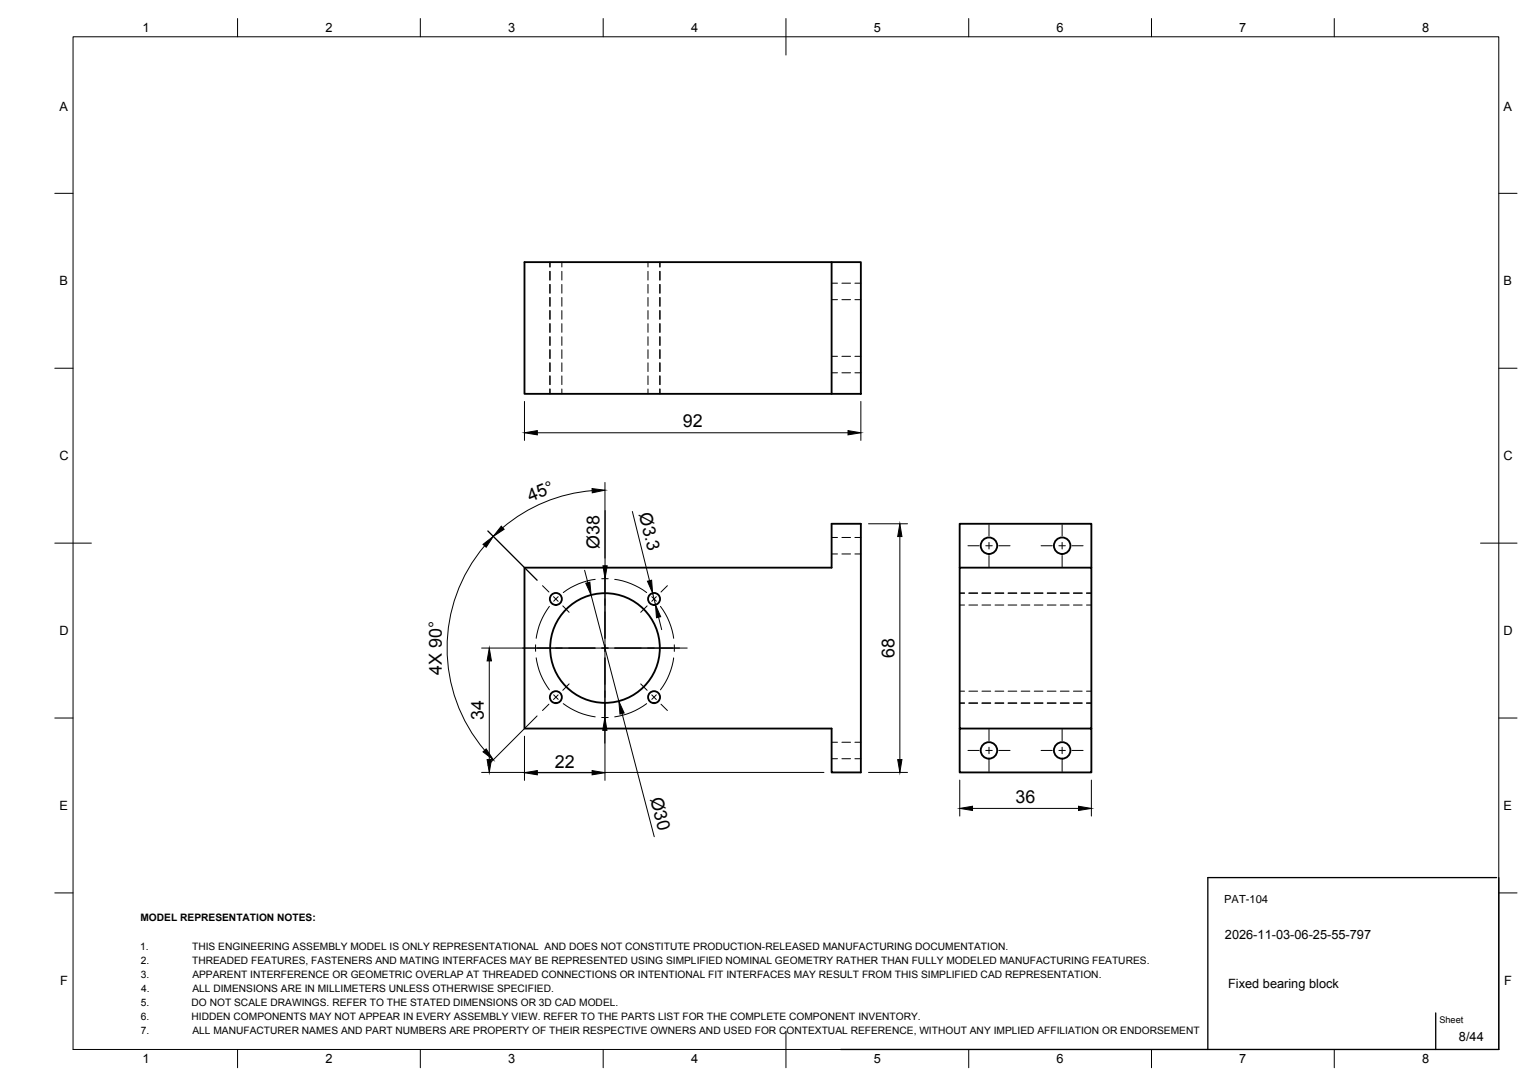
ISO-10303-21;
HEADER;
/* Generated by software containing ST-Developer
 * from STEP Tools, Inc. (www.steptools.com) 
 */

FILE_DESCRIPTION(
/* description */ ('Timing belt drive module 2 mm Pitch Timing 20T-40T'),

/* implementation_level */ '2;1');

FILE_NAME(
/* name */ 'Fixed bearing block.step',
/* time_stamp */ '2026-10-28T03:25:12-07:00',
/* author */ (''),
/* organization */ (''),
/* preprocessor_version */ 'ST-DEVELOPER v20.2',
/* originating_system */ 'Autodesk Translation Framework v15.17.0.0',
/* authorisation */ '');

FILE_SCHEMA (('AUTOMOTIVE_DESIGN { 1 0 10303 214 3 1 1 }'));
ENDSEC;

DATA;
#10=MECHANICAL_DESIGN_GEOMETRIC_PRESENTATION_REPRESENTATION('',(#527),#17830);
#441=SHAPE_REPRESENTATION_RELATIONSHIP('SRR','None',#18011,#484);
#484=ADVANCED_BREP_SHAPE_REPRESENTATION('',(#585),#17786);
#527=STYLED_ITEM('',(#18317),#585);
#585=MANIFOLD_SOLID_BREP('Body1',#8984);
#647=FACE_BOUND('',#1545,.T.);
#648=FACE_BOUND('',#1546,.T.);
#649=FACE_BOUND('',#1548,.T.);
#650=FACE_BOUND('',#1549,.T.);
#651=FACE_BOUND('',#1553,.T.);
#652=FACE_BOUND('',#1554,.T.);
#653=FACE_BOUND('',#1555,.T.);
#654=FACE_BOUND('',#1556,.T.);
#655=FACE_BOUND('',#1557,.T.);
#656=FACE_BOUND('',#1560,.T.);
#657=FACE_BOUND('',#1561,.T.);
#658=FACE_BOUND('',#1562,.T.);
#659=FACE_BOUND('',#1563,.T.);
#660=FACE_BOUND('',#1564,.T.);
#661=FACE_BOUND('',#1568,.T.);
#662=FACE_BOUND('',#1569,.T.);
#663=FACE_BOUND('',#1570,.T.);
#664=FACE_BOUND('',#1571,.T.);
#803=PLANE('',#9619);
#804=PLANE('',#9620);
#805=PLANE('',#9621);
#806=PLANE('',#9622);
#807=PLANE('',#9623);
#808=PLANE('',#9624);
#809=PLANE('',#9625);
#810=PLANE('',#9626);
#811=PLANE('',#9627);
#812=PLANE('',#9628);
#1004=FACE_OUTER_BOUND('',#1535,.T.);
#1005=FACE_OUTER_BOUND('',#1536,.T.);
#1006=FACE_OUTER_BOUND('',#1537,.T.);
#1007=FACE_OUTER_BOUND('',#1538,.T.);
#1008=FACE_OUTER_BOUND('',#1539,.T.);
#1009=FACE_OUTER_BOUND('',#1540,.T.);
#1010=FACE_OUTER_BOUND('',#1541,.T.);
#1011=FACE_OUTER_BOUND('',#1542,.T.);
#1012=FACE_OUTER_BOUND('',#1543,.T.);
#1013=FACE_OUTER_BOUND('',#1544,.T.);
#1014=FACE_OUTER_BOUND('',#1547,.T.);
#1015=FACE_OUTER_BOUND('',#1550,.T.);
#1016=FACE_OUTER_BOUND('',#1551,.T.);
#1017=FACE_OUTER_BOUND('',#1552,.T.);
#1018=FACE_OUTER_BOUND('',#1558,.T.);
#1019=FACE_OUTER_BOUND('',#1559,.T.);
#1020=FACE_OUTER_BOUND('',#1565,.T.);
#1021=FACE_OUTER_BOUND('',#1566,.T.);
#1022=FACE_OUTER_BOUND('',#1567,.T.);
#1535=EDGE_LOOP('',(#5977,#5978,#5979,#5980));
#1536=EDGE_LOOP('',(#5981,#5982,#5983,#5984));
#1537=EDGE_LOOP('',(#5985,#5986,#5987,#5988));
#1538=EDGE_LOOP('',(#5989,#5990,#5991,#5992));
#1539=EDGE_LOOP('',(#5993,#5994,#5995,#5996));
#1540=EDGE_LOOP('',(#5997,#5998,#5999,#6000));
#1541=EDGE_LOOP('',(#6001,#6002,#6003,#6004));
#1542=EDGE_LOOP('',(#6005,#6006,#6007,#6008));
#1543=EDGE_LOOP('',(#6009,#6010,#6011,#6012));
#1544=EDGE_LOOP('',(#6013,#6014,#6015,#6016));
#1545=EDGE_LOOP('',(#6017));
#1546=EDGE_LOOP('',(#6018));
#1547=EDGE_LOOP('',(#6019,#6020,#6021,#6022));
#1548=EDGE_LOOP('',(#6023));
#1549=EDGE_LOOP('',(#6024));
#1550=EDGE_LOOP('',(#6025,#6026,#6027,#6028));
#1551=EDGE_LOOP('',(#6029,#6030,#6031,#6032));
#1552=EDGE_LOOP('',(#6033,#6034,#6035,#6036,#6037,#6038,#6039,#6040));
#1553=EDGE_LOOP('',(#6041));
#1554=EDGE_LOOP('',(#6042));
#1555=EDGE_LOOP('',(#6043));
#1556=EDGE_LOOP('',(#6044));
#1557=EDGE_LOOP('',(#6045));
#1558=EDGE_LOOP('',(#6046,#6047,#6048,#6049));
#1559=EDGE_LOOP('',(#6050,#6051,#6052,#6053,#6054,#6055,#6056,#6057));
#1560=EDGE_LOOP('',(#6058));
#1561=EDGE_LOOP('',(#6059));
#1562=EDGE_LOOP('',(#6060));
#1563=EDGE_LOOP('',(#6061));
#1564=EDGE_LOOP('',(#6062));
#1565=EDGE_LOOP('',(#6063,#6064,#6065,#6066));
#1566=EDGE_LOOP('',(#6067,#6068,#6069,#6070));
#1567=EDGE_LOOP('',(#6071,#6072,#6073,#6074));
#1568=EDGE_LOOP('',(#6075));
#1569=EDGE_LOOP('',(#6076));
#1570=EDGE_LOOP('',(#6077));
#1571=EDGE_LOOP('',(#6078));
#2168=CIRCLE('',#9593,0.165);
#2169=CIRCLE('',#9594,0.165);
#2170=CIRCLE('',#9596,0.165);
#2171=CIRCLE('',#9597,0.165);
#2172=CIRCLE('',#9599,0.165);
#2173=CIRCLE('',#9600,0.165);
#2174=CIRCLE('',#9602,0.165);
#2175=CIRCLE('',#9603,0.165);
#2176=CIRCLE('',#9605,1.5);
#2177=CIRCLE('',#9606,1.5);
#2178=CIRCLE('',#9608,0.225);
#2179=CIRCLE('',#9609,0.225);
#2180=CIRCLE('',#9611,0.225);
#2181=CIRCLE('',#9612,0.225);
#2182=CIRCLE('',#9614,0.225);
#2183=CIRCLE('',#9615,0.225);
#2184=CIRCLE('',#9617,0.225);
#2185=CIRCLE('',#9618,0.225);
#2864=LINE('',#14095,#3342);
#2865=LINE('',#14101,#3343);
#2866=LINE('',#14107,#3344);
#2867=LINE('',#14113,#3345);
#2868=LINE('',#14119,#3346);
#2869=LINE('',#14125,#3347);
#2870=LINE('',#14131,#3348);
#2871=LINE('',#14137,#3349);
#2872=LINE('',#14143,#3350);
#2873=LINE('',#14148,#3351);
#2874=LINE('',#14150,#3352);
#2875=LINE('',#14152,#3353);
#2876=LINE('',#14153,#3354);
#2877=LINE('',#14157,#3355);
#2878=LINE('',#14159,#3356);
#2879=LINE('',#14161,#3357);
#2880=LINE('',#14162,#3358);
#2881=LINE('',#14165,#3359);
#2882=LINE('',#14167,#3360);
#2883=LINE('',#14168,#3361);
#2884=LINE('',#14171,#3362);
#2885=LINE('',#14173,#3363);
#2886=LINE('',#14174,#3364);
#2887=LINE('',#14177,#3365);
#2888=LINE('',#14179,#3366);
#2889=LINE('',#14180,#3367);
#2890=LINE('',#14181,#3368);
#2891=LINE('',#14184,#3369);
#2892=LINE('',#14185,#3370);
#2893=LINE('',#14188,#3371);
#2894=LINE('',#14189,#3372);
#2895=LINE('',#14190,#3373);
#2896=LINE('',#14192,#3374);
#3342=VECTOR('',#11039,0.165);
#3343=VECTOR('',#11046,0.165);
#3344=VECTOR('',#11053,0.165);
#3345=VECTOR('',#11060,0.165);
#3346=VECTOR('',#11067,1.5);
#3347=VECTOR('',#11074,0.225);
#3348=VECTOR('',#11081,0.225);
#3349=VECTOR('',#11088,0.225);
#3350=VECTOR('',#11095,0.225);
#3351=VECTOR('',#11100,1.);
#3352=VECTOR('',#11101,1.);
#3353=VECTOR('',#11102,1.);
#3354=VECTOR('',#11103,1.);
#3355=VECTOR('',#11106,1.);
#3356=VECTOR('',#11107,1.);
#3357=VECTOR('',#11108,1.);
#3358=VECTOR('',#11109,1.);
#3359=VECTOR('',#11112,1.);
#3360=VECTOR('',#11113,1.);
#3361=VECTOR('',#11114,1.);
#3362=VECTOR('',#11117,1.);
#3363=VECTOR('',#11118,1.);
#3364=VECTOR('',#11119,1.);
#3365=VECTOR('',#11122,1.);
#3366=VECTOR('',#11123,1.);
#3367=VECTOR('',#11124,1.);
#3368=VECTOR('',#11125,1.);
#3369=VECTOR('',#11128,1.);
#3370=VECTOR('',#11129,1.);
#3371=VECTOR('',#11132,1.);
#3372=VECTOR('',#11133,1.);
#3373=VECTOR('',#11134,1.);
#3374=VECTOR('',#11137,1.);
#3814=VERTEX_POINT('',#14092);
#3815=VERTEX_POINT('',#14094);
#3816=VERTEX_POINT('',#14098);
#3817=VERTEX_POINT('',#14100);
#3818=VERTEX_POINT('',#14104);
#3819=VERTEX_POINT('',#14106);
#3820=VERTEX_POINT('',#14110);
#3821=VERTEX_POINT('',#14112);
#3822=VERTEX_POINT('',#14116);
#3823=VERTEX_POINT('',#14118);
#3824=VERTEX_POINT('',#14122);
#3825=VERTEX_POINT('',#14124);
#3826=VERTEX_POINT('',#14128);
#3827=VERTEX_POINT('',#14130);
#3828=VERTEX_POINT('',#14134);
#3829=VERTEX_POINT('',#14136);
#3830=VERTEX_POINT('',#14140);
#3831=VERTEX_POINT('',#14142);
#3832=VERTEX_POINT('',#14146);
#3833=VERTEX_POINT('',#14147);
#3834=VERTEX_POINT('',#14149);
#3835=VERTEX_POINT('',#14151);
#3836=VERTEX_POINT('',#14155);
#3837=VERTEX_POINT('',#14156);
#3838=VERTEX_POINT('',#14158);
#3839=VERTEX_POINT('',#14160);
#3840=VERTEX_POINT('',#14164);
#3841=VERTEX_POINT('',#14166);
#3842=VERTEX_POINT('',#14170);
#3843=VERTEX_POINT('',#14172);
#3844=VERTEX_POINT('',#14176);
#3845=VERTEX_POINT('',#14178);
#3846=VERTEX_POINT('',#14183);
#3847=VERTEX_POINT('',#14187);
#4671=EDGE_CURVE('',#3814,#3814,#2168,.T.);
#4672=EDGE_CURVE('',#3814,#3815,#2864,.T.);
#4673=EDGE_CURVE('',#3815,#3815,#2169,.T.);
#4674=EDGE_CURVE('',#3816,#3816,#2170,.T.);
#4675=EDGE_CURVE('',#3816,#3817,#2865,.T.);
#4676=EDGE_CURVE('',#3817,#3817,#2171,.T.);
#4677=EDGE_CURVE('',#3818,#3818,#2172,.T.);
#4678=EDGE_CURVE('',#3818,#3819,#2866,.T.);
#4679=EDGE_CURVE('',#3819,#3819,#2173,.T.);
#4680=EDGE_CURVE('',#3820,#3820,#2174,.T.);
#4681=EDGE_CURVE('',#3820,#3821,#2867,.T.);
#4682=EDGE_CURVE('',#3821,#3821,#2175,.T.);
#4683=EDGE_CURVE('',#3822,#3822,#2176,.T.);
#4684=EDGE_CURVE('',#3822,#3823,#2868,.T.);
#4685=EDGE_CURVE('',#3823,#3823,#2177,.T.);
#4686=EDGE_CURVE('',#3824,#3824,#2178,.T.);
#4687=EDGE_CURVE('',#3824,#3825,#2869,.T.);
#4688=EDGE_CURVE('',#3825,#3825,#2179,.T.);
#4689=EDGE_CURVE('',#3826,#3826,#2180,.T.);
#4690=EDGE_CURVE('',#3826,#3827,#2870,.T.);
#4691=EDGE_CURVE('',#3827,#3827,#2181,.T.);
#4692=EDGE_CURVE('',#3828,#3828,#2182,.T.);
#4693=EDGE_CURVE('',#3828,#3829,#2871,.T.);
#4694=EDGE_CURVE('',#3829,#3829,#2183,.T.);
#4695=EDGE_CURVE('',#3830,#3830,#2184,.T.);
#4696=EDGE_CURVE('',#3830,#3831,#2872,.T.);
#4697=EDGE_CURVE('',#3831,#3831,#2185,.T.);
#4698=EDGE_CURVE('',#3832,#3833,#2873,.T.);
#4699=EDGE_CURVE('',#3834,#3832,#2874,.T.);
#4700=EDGE_CURVE('',#3834,#3835,#2875,.T.);
#4701=EDGE_CURVE('',#3833,#3835,#2876,.T.);
#4702=EDGE_CURVE('',#3836,#3837,#2877,.T.);
#4703=EDGE_CURVE('',#3838,#3836,#2878,.T.);
#4704=EDGE_CURVE('',#3839,#3838,#2879,.T.);
#4705=EDGE_CURVE('',#3837,#3839,#2880,.T.);
#4706=EDGE_CURVE('',#3839,#3840,#2881,.T.);
#4707=EDGE_CURVE('',#3841,#3838,#2882,.T.);
#4708=EDGE_CURVE('',#3840,#3841,#2883,.T.);
#4709=EDGE_CURVE('',#3842,#3834,#2884,.T.);
#4710=EDGE_CURVE('',#3842,#3843,#2885,.T.);
#4711=EDGE_CURVE('',#3835,#3843,#2886,.T.);
#4712=EDGE_CURVE('',#3832,#3844,#2887,.T.);
#4713=EDGE_CURVE('',#3845,#3844,#2888,.T.);
#4714=EDGE_CURVE('',#3837,#3845,#2889,.T.);
#4715=EDGE_CURVE('',#3840,#3842,#2890,.T.);
#4716=EDGE_CURVE('',#3833,#3846,#2891,.T.);
#4717=EDGE_CURVE('',#3844,#3846,#2892,.T.);
#4718=EDGE_CURVE('',#3836,#3847,#2893,.T.);
#4719=EDGE_CURVE('',#3846,#3847,#2894,.T.);
#4720=EDGE_CURVE('',#3843,#3841,#2895,.T.);
#4721=EDGE_CURVE('',#3847,#3845,#2896,.T.);
#5977=ORIENTED_EDGE('',*,*,#4671,.F.);
#5978=ORIENTED_EDGE('',*,*,#4672,.T.);
#5979=ORIENTED_EDGE('',*,*,#4673,.F.);
#5980=ORIENTED_EDGE('',*,*,#4672,.F.);
#5981=ORIENTED_EDGE('',*,*,#4674,.F.);
#5982=ORIENTED_EDGE('',*,*,#4675,.T.);
#5983=ORIENTED_EDGE('',*,*,#4676,.F.);
#5984=ORIENTED_EDGE('',*,*,#4675,.F.);
#5985=ORIENTED_EDGE('',*,*,#4677,.F.);
#5986=ORIENTED_EDGE('',*,*,#4678,.T.);
#5987=ORIENTED_EDGE('',*,*,#4679,.F.);
#5988=ORIENTED_EDGE('',*,*,#4678,.F.);
#5989=ORIENTED_EDGE('',*,*,#4680,.F.);
#5990=ORIENTED_EDGE('',*,*,#4681,.T.);
#5991=ORIENTED_EDGE('',*,*,#4682,.F.);
#5992=ORIENTED_EDGE('',*,*,#4681,.F.);
#5993=ORIENTED_EDGE('',*,*,#4683,.F.);
#5994=ORIENTED_EDGE('',*,*,#4684,.T.);
#5995=ORIENTED_EDGE('',*,*,#4685,.F.);
#5996=ORIENTED_EDGE('',*,*,#4684,.F.);
#5997=ORIENTED_EDGE('',*,*,#4686,.F.);
#5998=ORIENTED_EDGE('',*,*,#4687,.T.);
#5999=ORIENTED_EDGE('',*,*,#4688,.F.);
#6000=ORIENTED_EDGE('',*,*,#4687,.F.);
#6001=ORIENTED_EDGE('',*,*,#4689,.F.);
#6002=ORIENTED_EDGE('',*,*,#4690,.T.);
#6003=ORIENTED_EDGE('',*,*,#4691,.F.);
#6004=ORIENTED_EDGE('',*,*,#4690,.F.);
#6005=ORIENTED_EDGE('',*,*,#4692,.F.);
#6006=ORIENTED_EDGE('',*,*,#4693,.T.);
#6007=ORIENTED_EDGE('',*,*,#4694,.F.);
#6008=ORIENTED_EDGE('',*,*,#4693,.F.);
#6009=ORIENTED_EDGE('',*,*,#4695,.F.);
#6010=ORIENTED_EDGE('',*,*,#4696,.T.);
#6011=ORIENTED_EDGE('',*,*,#4697,.F.);
#6012=ORIENTED_EDGE('',*,*,#4696,.F.);
#6013=ORIENTED_EDGE('',*,*,#4698,.F.);
#6014=ORIENTED_EDGE('',*,*,#4699,.F.);
#6015=ORIENTED_EDGE('',*,*,#4700,.T.);
#6016=ORIENTED_EDGE('',*,*,#4701,.F.);
#6017=ORIENTED_EDGE('',*,*,#4688,.T.);
#6018=ORIENTED_EDGE('',*,*,#4697,.T.);
#6019=ORIENTED_EDGE('',*,*,#4702,.F.);
#6020=ORIENTED_EDGE('',*,*,#4703,.F.);
#6021=ORIENTED_EDGE('',*,*,#4704,.F.);
#6022=ORIENTED_EDGE('',*,*,#4705,.F.);
#6023=ORIENTED_EDGE('',*,*,#4691,.T.);
#6024=ORIENTED_EDGE('',*,*,#4694,.T.);
#6025=ORIENTED_EDGE('',*,*,#4706,.F.);
#6026=ORIENTED_EDGE('',*,*,#4704,.T.);
#6027=ORIENTED_EDGE('',*,*,#4707,.F.);
#6028=ORIENTED_EDGE('',*,*,#4708,.F.);
#6029=ORIENTED_EDGE('',*,*,#4709,.F.);
#6030=ORIENTED_EDGE('',*,*,#4710,.T.);
#6031=ORIENTED_EDGE('',*,*,#4711,.F.);
#6032=ORIENTED_EDGE('',*,*,#4700,.F.);
#6033=ORIENTED_EDGE('',*,*,#4712,.T.);
#6034=ORIENTED_EDGE('',*,*,#4713,.F.);
#6035=ORIENTED_EDGE('',*,*,#4714,.F.);
#6036=ORIENTED_EDGE('',*,*,#4705,.T.);
#6037=ORIENTED_EDGE('',*,*,#4706,.T.);
#6038=ORIENTED_EDGE('',*,*,#4715,.T.);
#6039=ORIENTED_EDGE('',*,*,#4709,.T.);
#6040=ORIENTED_EDGE('',*,*,#4699,.T.);
#6041=ORIENTED_EDGE('',*,*,#4683,.T.);
#6042=ORIENTED_EDGE('',*,*,#4680,.T.);
#6043=ORIENTED_EDGE('',*,*,#4677,.T.);
#6044=ORIENTED_EDGE('',*,*,#4674,.T.);
#6045=ORIENTED_EDGE('',*,*,#4671,.T.);
#6046=ORIENTED_EDGE('',*,*,#4698,.T.);
#6047=ORIENTED_EDGE('',*,*,#4716,.T.);
#6048=ORIENTED_EDGE('',*,*,#4717,.F.);
#6049=ORIENTED_EDGE('',*,*,#4712,.F.);
#6050=ORIENTED_EDGE('',*,*,#4718,.T.);
#6051=ORIENTED_EDGE('',*,*,#4719,.F.);
#6052=ORIENTED_EDGE('',*,*,#4716,.F.);
#6053=ORIENTED_EDGE('',*,*,#4701,.T.);
#6054=ORIENTED_EDGE('',*,*,#4711,.T.);
#6055=ORIENTED_EDGE('',*,*,#4720,.T.);
#6056=ORIENTED_EDGE('',*,*,#4707,.T.);
#6057=ORIENTED_EDGE('',*,*,#4703,.T.);
#6058=ORIENTED_EDGE('',*,*,#4685,.T.);
#6059=ORIENTED_EDGE('',*,*,#4682,.T.);
#6060=ORIENTED_EDGE('',*,*,#4679,.T.);
#6061=ORIENTED_EDGE('',*,*,#4676,.T.);
#6062=ORIENTED_EDGE('',*,*,#4673,.T.);
#6063=ORIENTED_EDGE('',*,*,#4702,.T.);
#6064=ORIENTED_EDGE('',*,*,#4714,.T.);
#6065=ORIENTED_EDGE('',*,*,#4721,.F.);
#6066=ORIENTED_EDGE('',*,*,#4718,.F.);
#6067=ORIENTED_EDGE('',*,*,#4721,.T.);
#6068=ORIENTED_EDGE('',*,*,#4713,.T.);
#6069=ORIENTED_EDGE('',*,*,#4717,.T.);
#6070=ORIENTED_EDGE('',*,*,#4719,.T.);
#6071=ORIENTED_EDGE('',*,*,#4720,.F.);
#6072=ORIENTED_EDGE('',*,*,#4710,.F.);
#6073=ORIENTED_EDGE('',*,*,#4715,.F.);
#6074=ORIENTED_EDGE('',*,*,#4708,.T.);
#6075=ORIENTED_EDGE('',*,*,#4686,.T.);
#6076=ORIENTED_EDGE('',*,*,#4689,.T.);
#6077=ORIENTED_EDGE('',*,*,#4692,.T.);
#6078=ORIENTED_EDGE('',*,*,#4695,.T.);
#8193=CYLINDRICAL_SURFACE('',#9592,0.165);
#8194=CYLINDRICAL_SURFACE('',#9595,0.165);
#8195=CYLINDRICAL_SURFACE('',#9598,0.165);
#8196=CYLINDRICAL_SURFACE('',#9601,0.165);
#8197=CYLINDRICAL_SURFACE('',#9604,1.5);
#8198=CYLINDRICAL_SURFACE('',#9607,0.225);
#8199=CYLINDRICAL_SURFACE('',#9610,0.225);
#8200=CYLINDRICAL_SURFACE('',#9613,0.225);
#8201=CYLINDRICAL_SURFACE('',#9616,0.225);
#8502=ADVANCED_FACE('',(#1004),#8193,.F.);
#8503=ADVANCED_FACE('',(#1005),#8194,.F.);
#8504=ADVANCED_FACE('',(#1006),#8195,.F.);
#8505=ADVANCED_FACE('',(#1007),#8196,.F.);
#8506=ADVANCED_FACE('',(#1008),#8197,.F.);
#8507=ADVANCED_FACE('',(#1009),#8198,.F.);
#8508=ADVANCED_FACE('',(#1010),#8199,.F.);
#8509=ADVANCED_FACE('',(#1011),#8200,.F.);
#8510=ADVANCED_FACE('',(#1012),#8201,.F.);
#8511=ADVANCED_FACE('',(#1013,#647,#648),#803,.T.);
#8512=ADVANCED_FACE('',(#1014,#649,#650),#804,.T.);
#8513=ADVANCED_FACE('',(#1015),#805,.T.);
#8514=ADVANCED_FACE('',(#1016),#806,.T.);
#8515=ADVANCED_FACE('',(#1017,#651,#652,#653,#654,#655),#807,.T.);
#8516=ADVANCED_FACE('',(#1018),#808,.T.);
#8517=ADVANCED_FACE('',(#1019,#656,#657,#658,#659,#660),#809,.T.);
#8518=ADVANCED_FACE('',(#1020),#810,.T.);
#8519=ADVANCED_FACE('',(#1021),#811,.T.);
#8520=ADVANCED_FACE('',(#1022,#661,#662,#663,#664),#812,.F.);
#8984=CLOSED_SHELL('',(#8502,#8503,#8504,#8505,#8506,#8507,#8508,#8509,
#8510,#8511,#8512,#8513,#8514,#8515,#8516,#8517,#8518,#8519,#8520));
#9591=AXIS2_PLACEMENT_3D('',#14090,#11033,#11034);
#9592=AXIS2_PLACEMENT_3D('',#14091,#11035,#11036);
#9593=AXIS2_PLACEMENT_3D('',#14093,#11037,#11038);
#9594=AXIS2_PLACEMENT_3D('',#14096,#11040,#11041);
#9595=AXIS2_PLACEMENT_3D('',#14097,#11042,#11043);
#9596=AXIS2_PLACEMENT_3D('',#14099,#11044,#11045);
#9597=AXIS2_PLACEMENT_3D('',#14102,#11047,#11048);
#9598=AXIS2_PLACEMENT_3D('',#14103,#11049,#11050);
#9599=AXIS2_PLACEMENT_3D('',#14105,#11051,#11052);
#9600=AXIS2_PLACEMENT_3D('',#14108,#11054,#11055);
#9601=AXIS2_PLACEMENT_3D('',#14109,#11056,#11057);
#9602=AXIS2_PLACEMENT_3D('',#14111,#11058,#11059);
#9603=AXIS2_PLACEMENT_3D('',#14114,#11061,#11062);
#9604=AXIS2_PLACEMENT_3D('',#14115,#11063,#11064);
#9605=AXIS2_PLACEMENT_3D('',#14117,#11065,#11066);
#9606=AXIS2_PLACEMENT_3D('',#14120,#11068,#11069);
#9607=AXIS2_PLACEMENT_3D('',#14121,#11070,#11071);
#9608=AXIS2_PLACEMENT_3D('',#14123,#11072,#11073);
#9609=AXIS2_PLACEMENT_3D('',#14126,#11075,#11076);
#9610=AXIS2_PLACEMENT_3D('',#14127,#11077,#11078);
#9611=AXIS2_PLACEMENT_3D('',#14129,#11079,#11080);
#9612=AXIS2_PLACEMENT_3D('',#14132,#11082,#11083);
#9613=AXIS2_PLACEMENT_3D('',#14133,#11084,#11085);
#9614=AXIS2_PLACEMENT_3D('',#14135,#11086,#11087);
#9615=AXIS2_PLACEMENT_3D('',#14138,#11089,#11090);
#9616=AXIS2_PLACEMENT_3D('',#14139,#11091,#11092);
#9617=AXIS2_PLACEMENT_3D('',#14141,#11093,#11094);
#9618=AXIS2_PLACEMENT_3D('',#14144,#11096,#11097);
#9619=AXIS2_PLACEMENT_3D('',#14145,#11098,#11099);
#9620=AXIS2_PLACEMENT_3D('',#14154,#11104,#11105);
#9621=AXIS2_PLACEMENT_3D('',#14163,#11110,#11111);
#9622=AXIS2_PLACEMENT_3D('',#14169,#11115,#11116);
#9623=AXIS2_PLACEMENT_3D('',#14175,#11120,#11121);
#9624=AXIS2_PLACEMENT_3D('',#14182,#11126,#11127);
#9625=AXIS2_PLACEMENT_3D('',#14186,#11130,#11131);
#9626=AXIS2_PLACEMENT_3D('',#14191,#11135,#11136);
#9627=AXIS2_PLACEMENT_3D('',#14193,#11138,#11139);
#9628=AXIS2_PLACEMENT_3D('',#14194,#11140,#11141);
#11033=DIRECTION('axis',(0.,0.,1.));
#11034=DIRECTION('refdir',(1.,0.,0.));
#11035=DIRECTION('center_axis',(0.,1.,0.));
#11036=DIRECTION('ref_axis',(1.,0.,0.));
#11037=DIRECTION('center_axis',(0.,1.,0.));
#11038=DIRECTION('ref_axis',(1.,0.,0.));
#11039=DIRECTION('',(0.,1.,0.));
#11040=DIRECTION('center_axis',(0.,-1.,0.));
#11041=DIRECTION('ref_axis',(1.,0.,0.));
#11042=DIRECTION('center_axis',(0.,1.,0.));
#11043=DIRECTION('ref_axis',(1.,0.,0.));
#11044=DIRECTION('center_axis',(0.,1.,0.));
#11045=DIRECTION('ref_axis',(1.,0.,0.));
#11046=DIRECTION('',(0.,1.,0.));
#11047=DIRECTION('center_axis',(0.,-1.,0.));
#11048=DIRECTION('ref_axis',(1.,0.,0.));
#11049=DIRECTION('center_axis',(0.,1.,0.));
#11050=DIRECTION('ref_axis',(1.,0.,0.));
#11051=DIRECTION('center_axis',(0.,1.,0.));
#11052=DIRECTION('ref_axis',(1.,0.,0.));
#11053=DIRECTION('',(0.,1.,0.));
#11054=DIRECTION('center_axis',(0.,-1.,0.));
#11055=DIRECTION('ref_axis',(1.,0.,0.));
#11056=DIRECTION('center_axis',(0.,1.,0.));
#11057=DIRECTION('ref_axis',(1.,0.,0.));
#11058=DIRECTION('center_axis',(0.,1.,0.));
#11059=DIRECTION('ref_axis',(1.,0.,0.));
#11060=DIRECTION('',(0.,1.,0.));
#11061=DIRECTION('center_axis',(0.,-1.,0.));
#11062=DIRECTION('ref_axis',(1.,0.,0.));
#11063=DIRECTION('center_axis',(0.,1.,0.));
#11064=DIRECTION('ref_axis',(1.,0.,0.));
#11065=DIRECTION('center_axis',(0.,1.,0.));
#11066=DIRECTION('ref_axis',(1.,0.,0.));
#11067=DIRECTION('',(0.,1.,0.));
#11068=DIRECTION('center_axis',(0.,-1.,0.));
#11069=DIRECTION('ref_axis',(1.,0.,0.));
#11070=DIRECTION('center_axis',(0.,0.,1.));
#11071=DIRECTION('ref_axis',(1.,0.,0.));
#11072=DIRECTION('center_axis',(0.,0.,1.));
#11073=DIRECTION('ref_axis',(1.,0.,0.));
#11074=DIRECTION('',(0.,0.,1.));
#11075=DIRECTION('center_axis',(0.,0.,-1.));
#11076=DIRECTION('ref_axis',(1.,0.,0.));
#11077=DIRECTION('center_axis',(0.,0.,1.));
#11078=DIRECTION('ref_axis',(1.,0.,0.));
#11079=DIRECTION('center_axis',(0.,0.,1.));
#11080=DIRECTION('ref_axis',(1.,0.,0.));
#11081=DIRECTION('',(0.,0.,1.));
#11082=DIRECTION('center_axis',(0.,0.,-1.));
#11083=DIRECTION('ref_axis',(1.,0.,0.));
#11084=DIRECTION('center_axis',(0.,0.,1.));
#11085=DIRECTION('ref_axis',(1.,0.,0.));
#11086=DIRECTION('center_axis',(0.,0.,1.));
#11087=DIRECTION('ref_axis',(1.,0.,0.));
#11088=DIRECTION('',(0.,0.,1.));
#11089=DIRECTION('center_axis',(0.,0.,-1.));
#11090=DIRECTION('ref_axis',(1.,0.,0.));
#11091=DIRECTION('center_axis',(0.,0.,1.));
#11092=DIRECTION('ref_axis',(1.,0.,0.));
#11093=DIRECTION('center_axis',(0.,0.,1.));
#11094=DIRECTION('ref_axis',(1.,0.,0.));
#11095=DIRECTION('',(0.,0.,1.));
#11096=DIRECTION('center_axis',(0.,0.,-1.));
#11097=DIRECTION('ref_axis',(1.,0.,0.));
#11098=DIRECTION('center_axis',(0.,0.,1.));
#11099=DIRECTION('ref_axis',(1.,0.,0.));
#11100=DIRECTION('',(0.,1.,0.));
#11101=DIRECTION('',(-1.,0.,0.));
#11102=DIRECTION('',(0.,1.,0.));
#11103=DIRECTION('',(1.,0.,0.));
#11104=DIRECTION('center_axis',(0.,0.,1.));
#11105=DIRECTION('ref_axis',(1.,0.,0.));
#11106=DIRECTION('',(0.,-1.,0.));
#11107=DIRECTION('',(1.,0.,0.));
#11108=DIRECTION('',(0.,1.,0.));
#11109=DIRECTION('',(-1.,0.,0.));
#11110=DIRECTION('center_axis',(-1.,0.,0.));
#11111=DIRECTION('ref_axis',(0.,0.,1.));
#11112=DIRECTION('',(0.,0.,-1.));
#11113=DIRECTION('',(0.,0.,1.));
#11114=DIRECTION('',(0.,1.,0.));
#11115=DIRECTION('center_axis',(1.,0.,0.));
#11116=DIRECTION('ref_axis',(0.,0.,-1.));
#11117=DIRECTION('',(0.,0.,1.));
#11118=DIRECTION('',(0.,1.,0.));
#11119=DIRECTION('',(0.,0.,-1.));
#11120=DIRECTION('center_axis',(0.,-1.,0.));
#11121=DIRECTION('ref_axis',(1.,0.,0.));
#11122=DIRECTION('',(0.,0.,1.));
#11123=DIRECTION('',(1.,0.,0.));
#11124=DIRECTION('',(0.,0.,1.));
#11125=DIRECTION('',(1.,0.,0.));
#11126=DIRECTION('center_axis',(1.,0.,0.));
#11127=DIRECTION('ref_axis',(0.,1.,0.));
#11128=DIRECTION('',(0.,0.,1.));
#11129=DIRECTION('',(0.,1.,0.));
#11130=DIRECTION('center_axis',(0.,1.,0.));
#11131=DIRECTION('ref_axis',(-1.,0.,0.));
#11132=DIRECTION('',(0.,0.,1.));
#11133=DIRECTION('',(-1.,0.,0.));
#11134=DIRECTION('',(-1.,0.,0.));
#11135=DIRECTION('center_axis',(-1.,0.,0.));
#11136=DIRECTION('ref_axis',(0.,-1.,0.));
#11137=DIRECTION('',(0.,-1.,0.));
#11138=DIRECTION('center_axis',(0.,0.,1.));
#11139=DIRECTION('ref_axis',(1.,0.,0.));
#11140=DIRECTION('center_axis',(0.,0.,1.));
#11141=DIRECTION('ref_axis',(1.,0.,0.));
#14090=CARTESIAN_POINT('',(0.,0.,0.));
#14091=CARTESIAN_POINT('Origin',(-1.34350288425444,-1.9,5.65649711574556));
#14092=CARTESIAN_POINT('',(-1.50850288425444,-1.8,5.65649711574556));
#14093=CARTESIAN_POINT('Origin',(-1.34350288425444,-1.8,5.65649711574556));
#14094=CARTESIAN_POINT('',(-1.50850288425444,1.8,5.65649711574556));
#14095=CARTESIAN_POINT('',(-1.50850288425444,-1.9,5.65649711574556));
#14096=CARTESIAN_POINT('Origin',(-1.34350288425444,1.8,5.65649711574556));
#14097=CARTESIAN_POINT('Origin',(-1.34350288425444,-1.9,8.34350288425444));
#14098=CARTESIAN_POINT('',(-1.50850288425444,-1.8,8.34350288425444));
#14099=CARTESIAN_POINT('Origin',(-1.34350288425444,-1.8,8.34350288425444));
#14100=CARTESIAN_POINT('',(-1.50850288425444,1.8,8.34350288425444));
#14101=CARTESIAN_POINT('',(-1.50850288425444,-1.9,8.34350288425444));
#14102=CARTESIAN_POINT('Origin',(-1.34350288425444,1.8,8.34350288425444));
#14103=CARTESIAN_POINT('Origin',(1.34350288425444,-1.9,8.34350288425444));
#14104=CARTESIAN_POINT('',(1.17850288425444,-1.8,8.34350288425444));
#14105=CARTESIAN_POINT('Origin',(1.34350288425444,-1.8,8.34350288425444));
#14106=CARTESIAN_POINT('',(1.17850288425444,1.8,8.34350288425444));
#14107=CARTESIAN_POINT('',(1.17850288425444,-1.9,8.34350288425444));
#14108=CARTESIAN_POINT('Origin',(1.34350288425444,1.8,8.34350288425444));
#14109=CARTESIAN_POINT('Origin',(1.34350288425444,-1.9,5.65649711574556));
#14110=CARTESIAN_POINT('',(1.17850288425444,-1.8,5.65649711574556));
#14111=CARTESIAN_POINT('Origin',(1.34350288425444,-1.8,5.65649711574556));
#14112=CARTESIAN_POINT('',(1.17850288425444,1.8,5.65649711574556));
#14113=CARTESIAN_POINT('',(1.17850288425444,-1.9,5.65649711574556));
#14114=CARTESIAN_POINT('Origin',(1.34350288425444,1.8,5.65649711574556));
#14115=CARTESIAN_POINT('Origin',(0.,-1.9,7.));
#14116=CARTESIAN_POINT('',(-1.5,-1.8,7.));
#14117=CARTESIAN_POINT('Origin',(0.,-1.8,7.));
#14118=CARTESIAN_POINT('',(-1.5,1.8,7.));
#14119=CARTESIAN_POINT('',(-1.5,-1.9,7.));
#14120=CARTESIAN_POINT('Origin',(0.,1.8,7.));
#14121=CARTESIAN_POINT('Origin',(2.8,-1.,-0.1));
#14122=CARTESIAN_POINT('',(2.575,-1.,0.));
#14123=CARTESIAN_POINT('Origin',(2.8,-1.,0.));
#14124=CARTESIAN_POINT('',(2.575,-1.,0.8));
#14125=CARTESIAN_POINT('',(2.575,-1.,-0.1));
#14126=CARTESIAN_POINT('Origin',(2.8,-1.,0.8));
#14127=CARTESIAN_POINT('Origin',(-2.8,1.,-0.1));
#14128=CARTESIAN_POINT('',(-3.025,1.,0.));
#14129=CARTESIAN_POINT('Origin',(-2.8,1.,0.));
#14130=CARTESIAN_POINT('',(-3.025,1.,0.8));
#14131=CARTESIAN_POINT('',(-3.025,1.,-0.1));
#14132=CARTESIAN_POINT('Origin',(-2.8,1.,0.8));
#14133=CARTESIAN_POINT('Origin',(-2.8,-1.,-0.1));
#14134=CARTESIAN_POINT('',(-3.025,-1.,0.));
#14135=CARTESIAN_POINT('Origin',(-2.8,-1.,0.));
#14136=CARTESIAN_POINT('',(-3.025,-1.,0.8));
#14137=CARTESIAN_POINT('',(-3.025,-1.,-0.1));
#14138=CARTESIAN_POINT('Origin',(-2.8,-1.,0.8));
#14139=CARTESIAN_POINT('Origin',(2.8,1.,-0.1));
#14140=CARTESIAN_POINT('',(2.575,1.,0.));
#14141=CARTESIAN_POINT('Origin',(2.8,1.,0.));
#14142=CARTESIAN_POINT('',(2.575,1.,0.8));
#14143=CARTESIAN_POINT('',(2.575,1.,-0.1));
#14144=CARTESIAN_POINT('Origin',(2.8,1.,0.8));
#14145=CARTESIAN_POINT('Origin',(-3.4,-1.8,0.8));
#14146=CARTESIAN_POINT('',(2.2,-1.8,0.8));
#14147=CARTESIAN_POINT('',(2.2,1.8,0.8));
#14148=CARTESIAN_POINT('',(2.2,-1.8,0.8));
#14149=CARTESIAN_POINT('',(3.4,-1.8,0.8));
#14150=CARTESIAN_POINT('',(3.4,-1.8,0.8));
#14151=CARTESIAN_POINT('',(3.4,1.8,0.8));
#14152=CARTESIAN_POINT('',(3.4,-1.8,0.8));
#14153=CARTESIAN_POINT('',(3.4,1.8,0.8));
#14154=CARTESIAN_POINT('Origin',(-3.4,-1.8,0.8));
#14155=CARTESIAN_POINT('',(-2.2,1.8,0.8));
#14156=CARTESIAN_POINT('',(-2.2,-1.8,0.8));
#14157=CARTESIAN_POINT('',(-2.2,0.,0.8));
#14158=CARTESIAN_POINT('',(-3.4,1.8,0.8));
#14159=CARTESIAN_POINT('',(3.4,1.8,0.8));
#14160=CARTESIAN_POINT('',(-3.4,-1.8,0.8));
#14161=CARTESIAN_POINT('',(-3.4,-1.8,0.8));
#14162=CARTESIAN_POINT('',(3.4,-1.8,0.8));
#14163=CARTESIAN_POINT('Origin',(-3.4,-1.8,0.));
#14164=CARTESIAN_POINT('',(-3.4,-1.8,0.));
#14165=CARTESIAN_POINT('',(-3.4,-1.8,0.8));
#14166=CARTESIAN_POINT('',(-3.4,1.8,0.));
#14167=CARTESIAN_POINT('',(-3.4,1.8,0.8));
#14168=CARTESIAN_POINT('',(-3.4,-1.8,0.));
#14169=CARTESIAN_POINT('Origin',(3.4,-1.8,0.8));
#14170=CARTESIAN_POINT('',(3.4,-1.8,0.));
#14171=CARTESIAN_POINT('',(3.4,-1.8,0.));
#14172=CARTESIAN_POINT('',(3.4,1.8,0.));
#14173=CARTESIAN_POINT('',(3.4,-1.8,0.));
#14174=CARTESIAN_POINT('',(3.4,1.8,0.));
#14175=CARTESIAN_POINT('Origin',(-2.2,-1.8,0.));
#14176=CARTESIAN_POINT('',(2.2,-1.8,9.2));
#14177=CARTESIAN_POINT('',(2.2,-1.8,0.));
#14178=CARTESIAN_POINT('',(-2.2,-1.8,9.2));
#14179=CARTESIAN_POINT('',(-2.2,-1.8,9.2));
#14180=CARTESIAN_POINT('',(-2.2,-1.8,0.));
#14181=CARTESIAN_POINT('',(-3.4,-1.8,0.));
#14182=CARTESIAN_POINT('Origin',(2.2,-1.8,0.));
#14183=CARTESIAN_POINT('',(2.2,1.8,9.2));
#14184=CARTESIAN_POINT('',(2.2,1.8,0.));
#14185=CARTESIAN_POINT('',(2.2,-1.8,9.2));
#14186=CARTESIAN_POINT('Origin',(2.2,1.8,0.));
#14187=CARTESIAN_POINT('',(-2.2,1.8,9.2));
#14188=CARTESIAN_POINT('',(-2.2,1.8,0.));
#14189=CARTESIAN_POINT('',(2.2,1.8,9.2));
#14190=CARTESIAN_POINT('',(-3.4,1.8,0.));
#14191=CARTESIAN_POINT('Origin',(-2.2,1.8,0.));
#14192=CARTESIAN_POINT('',(-2.2,1.8,9.2));
#14193=CARTESIAN_POINT('Origin',(0.,0.,9.2));
#14194=CARTESIAN_POINT('Origin',(0.,0.,0.));
#17736=UNCERTAINTY_MEASURE_WITH_UNIT(LENGTH_MEASURE(0.001),#17831,
'DISTANCE_ACCURACY_VALUE',
'Maximum model space distance between geometric entities at asserted c
onnectivities');
#17780=UNCERTAINTY_MEASURE_WITH_UNIT(LENGTH_MEASURE(0.001),#17831,
'DISTANCE_ACCURACY_VALUE',
'Maximum model space distance between geometric entities at asserted c
onnectivities');
#17786=(
GEOMETRIC_REPRESENTATION_CONTEXT(3)
GLOBAL_UNCERTAINTY_ASSIGNED_CONTEXT((#17736))
GLOBAL_UNIT_ASSIGNED_CONTEXT((#17831,#17833,#17834))
REPRESENTATION_CONTEXT('','3D')
);
#17830=(
GEOMETRIC_REPRESENTATION_CONTEXT(3)
GLOBAL_UNCERTAINTY_ASSIGNED_CONTEXT((#17780))
GLOBAL_UNIT_ASSIGNED_CONTEXT((#17831,#17833,#17834))
REPRESENTATION_CONTEXT('','3D')
);
#17831=(
LENGTH_UNIT()
NAMED_UNIT(*)
SI_UNIT(.CENTI.,.METRE.)
);
#17833=(
NAMED_UNIT(*)
PLANE_ANGLE_UNIT()
SI_UNIT($,.RADIAN.)
);
#17834=(
NAMED_UNIT(*)
SI_UNIT($,.STERADIAN.)
SOLID_ANGLE_UNIT()
);
#17840=SHAPE_DEFINITION_REPRESENTATION(#17889,#18011);
#17889=PRODUCT_DEFINITION_SHAPE('',$,#18061);
#18011=SHAPE_REPRESENTATION('',(#9591),#17786);
#18055=PRODUCT_DEFINITION_CONTEXT('part definition',#18204,'design');
#18061=PRODUCT_DEFINITION('Fixed bearing block','Fixed bearing block',#18110,
#18055);
#18110=PRODUCT_DEFINITION_FORMATION('',$,#18211);
#18204=APPLICATION_CONTEXT(
'Core Data for Automotive Mechanical Design Process');
#18205=PRODUCT_CONTEXT('part definition',#18204,'mechanical');
#18211=PRODUCT('Fixed bearing block','Fixed bearing block',
'Fixed bearing block',(#18205));
#18311=COLOUR_RGB('Grey',0.48,0.52,0.57);
#18312=FILL_AREA_STYLE_COLOUR('',#18311);
#18313=FILL_AREA_STYLE('',(#18312));
#18314=SURFACE_STYLE_FILL_AREA(#18313);
#18315=SURFACE_SIDE_STYLE('',(#18314));
#18316=SURFACE_STYLE_USAGE(.BOTH.,#18315);
#18317=PRESENTATION_STYLE_ASSIGNMENT((#18316));
ENDSEC;
END-ISO-10303-21;
